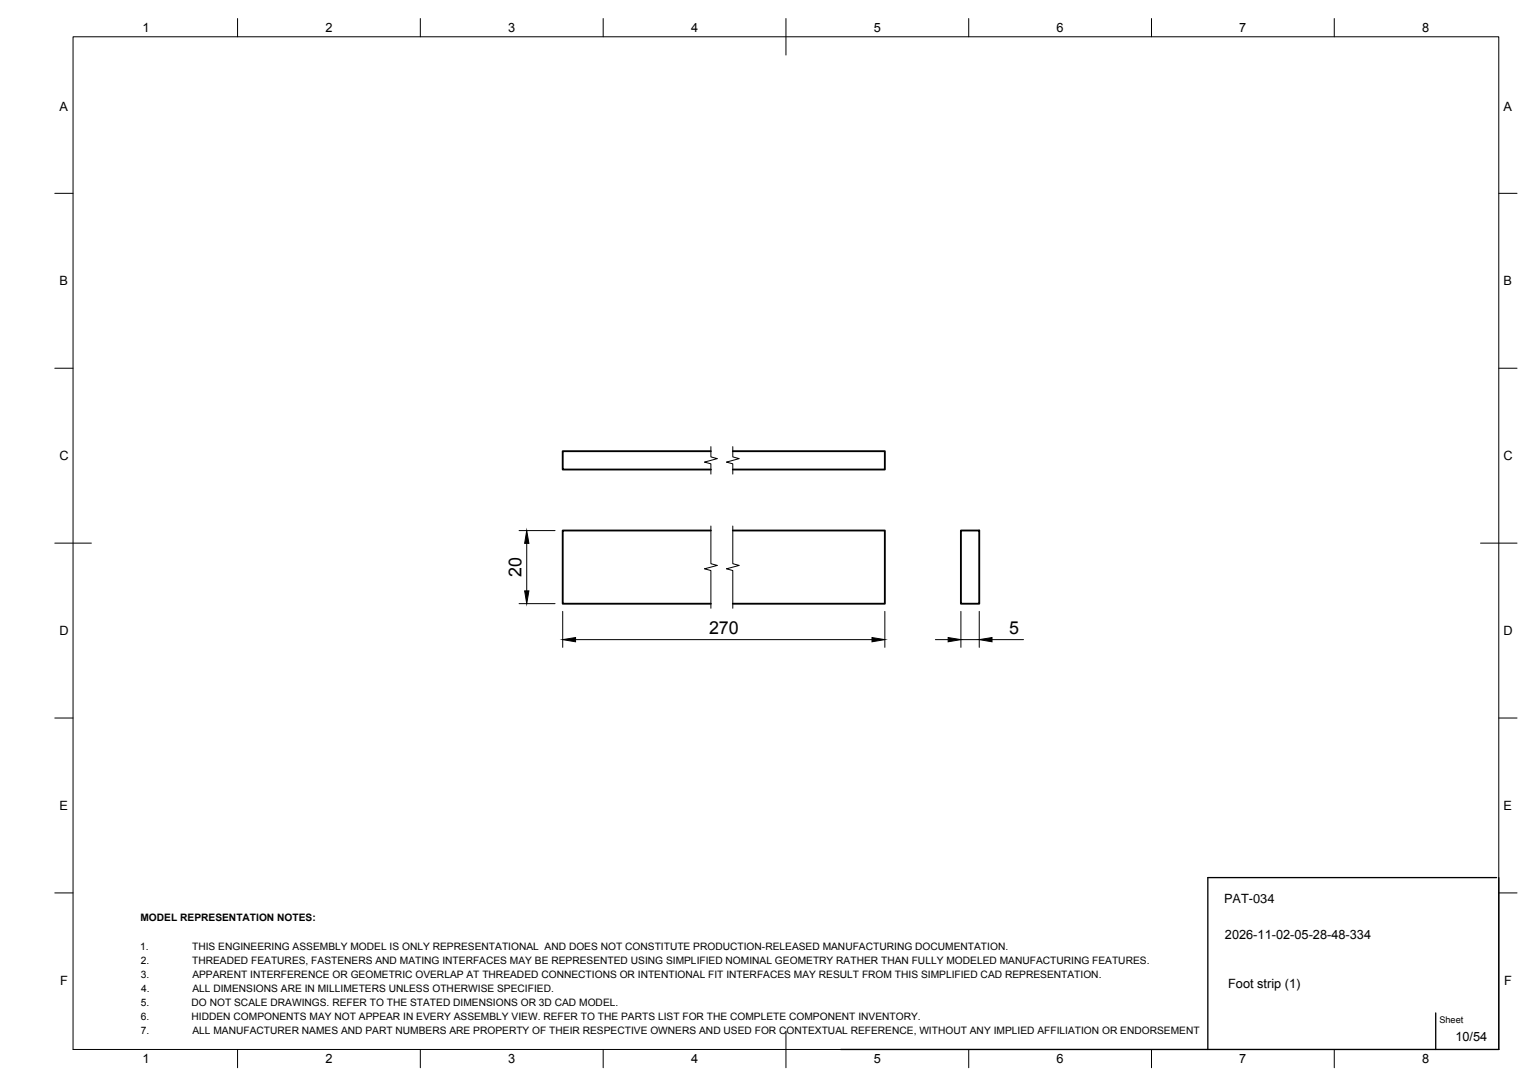
ISO-10303-21;
HEADER;
/* Generated by software containing ST-Developer
 * from STEP Tools, Inc. (www.steptools.com) 
 */

FILE_DESCRIPTION(
/* description */ ('Fatigue rig crank-slider'),
/* implementation_level */ '2;1');

FILE_NAME(
/* name */ 'Foot strip (1).step',
/* time_stamp */ '2026-10-28T03:24:50-07:00',
/* author */ (''),
/* organization */ (''),
/* preprocessor_version */ 'ST-DEVELOPER v20.2',
/* originating_system */ 'Autodesk Translation Framework v15.17.0.0',
/* authorisation */ '');

FILE_SCHEMA (('AUTOMOTIVE_DESIGN { 1 0 10303 214 3 1 1 }'));
ENDSEC;

DATA;
#10=MECHANICAL_DESIGN_GEOMETRIC_PRESENTATION_REPRESENTATION('',(#596),#16911);
#496=SHAPE_REPRESENTATION_RELATIONSHIP('SRR','None',#17135,#546);
#546=ADVANCED_BREP_SHAPE_REPRESENTATION('',(#655),#16864);
#596=STYLED_ITEM('',(#17473),#655);
#655=MANIFOLD_SOLID_BREP('Body1',#8887);
#955=PLANE('',#9719);
#956=PLANE('',#9720);
#957=PLANE('',#9721);
#958=PLANE('',#9722);
#959=PLANE('',#9723);
#960=PLANE('',#9724);
#1327=FACE_OUTER_BOUND('',#1926,.T.);
#1328=FACE_OUTER_BOUND('',#1927,.T.);
#1329=FACE_OUTER_BOUND('',#1928,.T.);
#1330=FACE_OUTER_BOUND('',#1929,.T.);
#1331=FACE_OUTER_BOUND('',#1930,.T.);
#1332=FACE_OUTER_BOUND('',#1931,.T.);
#1926=EDGE_LOOP('',(#6428,#6429,#6430,#6431));
#1927=EDGE_LOOP('',(#6432,#6433,#6434,#6435));
#1928=EDGE_LOOP('',(#6436,#6437,#6438,#6439));
#1929=EDGE_LOOP('',(#6440,#6441,#6442,#6443));
#1930=EDGE_LOOP('',(#6444,#6445,#6446,#6447));
#1931=EDGE_LOOP('',(#6448,#6449,#6450,#6451));
#2572=LINE('',#13843,#3218);
#2573=LINE('',#13845,#3219);
#2574=LINE('',#13847,#3220);
#2575=LINE('',#13848,#3221);
#2576=LINE('',#13851,#3222);
#2577=LINE('',#13853,#3223);
#2578=LINE('',#13854,#3224);
#2579=LINE('',#13857,#3225);
#2580=LINE('',#13859,#3226);
#2581=LINE('',#13860,#3227);
#2582=LINE('',#13862,#3228);
#2583=LINE('',#13863,#3229);
#3218=VECTOR('',#11132,1.);
#3219=VECTOR('',#11133,1.);
#3220=VECTOR('',#11134,1.);
#3221=VECTOR('',#11135,1.);
#3222=VECTOR('',#11138,1.);
#3223=VECTOR('',#11139,1.);
#3224=VECTOR('',#11140,1.);
#3225=VECTOR('',#11143,1.);
#3226=VECTOR('',#11144,1.);
#3227=VECTOR('',#11145,1.);
#3228=VECTOR('',#11148,1.);
#3229=VECTOR('',#11149,1.);
#4296=VERTEX_POINT('',#13841);
#4297=VERTEX_POINT('',#13842);
#4298=VERTEX_POINT('',#13844);
#4299=VERTEX_POINT('',#13846);
#4300=VERTEX_POINT('',#13850);
#4301=VERTEX_POINT('',#13852);
#4302=VERTEX_POINT('',#13856);
#4303=VERTEX_POINT('',#13858);
#5112=EDGE_CURVE('',#4296,#4297,#2572,.T.);
#5113=EDGE_CURVE('',#4297,#4298,#2573,.T.);
#5114=EDGE_CURVE('',#4299,#4298,#2574,.T.);
#5115=EDGE_CURVE('',#4296,#4299,#2575,.T.);
#5116=EDGE_CURVE('',#4300,#4296,#2576,.T.);
#5117=EDGE_CURVE('',#4301,#4299,#2577,.T.);
#5118=EDGE_CURVE('',#4300,#4301,#2578,.T.);
#5119=EDGE_CURVE('',#4302,#4300,#2579,.T.);
#5120=EDGE_CURVE('',#4303,#4301,#2580,.T.);
#5121=EDGE_CURVE('',#4302,#4303,#2581,.T.);
#5122=EDGE_CURVE('',#4297,#4302,#2582,.T.);
#5123=EDGE_CURVE('',#4298,#4303,#2583,.T.);
#6428=ORIENTED_EDGE('',*,*,#5112,.T.);
#6429=ORIENTED_EDGE('',*,*,#5113,.T.);
#6430=ORIENTED_EDGE('',*,*,#5114,.F.);
#6431=ORIENTED_EDGE('',*,*,#5115,.F.);
#6432=ORIENTED_EDGE('',*,*,#5116,.T.);
#6433=ORIENTED_EDGE('',*,*,#5115,.T.);
#6434=ORIENTED_EDGE('',*,*,#5117,.F.);
#6435=ORIENTED_EDGE('',*,*,#5118,.F.);
#6436=ORIENTED_EDGE('',*,*,#5119,.T.);
#6437=ORIENTED_EDGE('',*,*,#5118,.T.);
#6438=ORIENTED_EDGE('',*,*,#5120,.F.);
#6439=ORIENTED_EDGE('',*,*,#5121,.F.);
#6440=ORIENTED_EDGE('',*,*,#5122,.T.);
#6441=ORIENTED_EDGE('',*,*,#5121,.T.);
#6442=ORIENTED_EDGE('',*,*,#5123,.F.);
#6443=ORIENTED_EDGE('',*,*,#5113,.F.);
#6444=ORIENTED_EDGE('',*,*,#5123,.T.);
#6445=ORIENTED_EDGE('',*,*,#5120,.T.);
#6446=ORIENTED_EDGE('',*,*,#5117,.T.);
#6447=ORIENTED_EDGE('',*,*,#5114,.T.);
#6448=ORIENTED_EDGE('',*,*,#5122,.F.);
#6449=ORIENTED_EDGE('',*,*,#5112,.F.);
#6450=ORIENTED_EDGE('',*,*,#5116,.F.);
#6451=ORIENTED_EDGE('',*,*,#5119,.F.);
#8465=ADVANCED_FACE('',(#1327),#955,.T.);
#8466=ADVANCED_FACE('',(#1328),#956,.T.);
#8467=ADVANCED_FACE('',(#1329),#957,.T.);
#8468=ADVANCED_FACE('',(#1330),#958,.T.);
#8469=ADVANCED_FACE('',(#1331),#959,.T.);
#8470=ADVANCED_FACE('',(#1332),#960,.F.);
#8887=CLOSED_SHELL('',(#8465,#8466,#8467,#8468,#8469,#8470));
#9718=AXIS2_PLACEMENT_3D('',#13839,#11128,#11129);
#9719=AXIS2_PLACEMENT_3D('',#13840,#11130,#11131);
#9720=AXIS2_PLACEMENT_3D('',#13849,#11136,#11137);
#9721=AXIS2_PLACEMENT_3D('',#13855,#11141,#11142);
#9722=AXIS2_PLACEMENT_3D('',#13861,#11146,#11147);
#9723=AXIS2_PLACEMENT_3D('',#13864,#11150,#11151);
#9724=AXIS2_PLACEMENT_3D('',#13865,#11152,#11153);
#11128=DIRECTION('axis',(0.,0.,1.));
#11129=DIRECTION('refdir',(1.,0.,0.));
#11130=DIRECTION('center_axis',(0.,1.,0.));
#11131=DIRECTION('ref_axis',(-1.,0.,0.));
#11132=DIRECTION('',(-1.,0.,0.));
#11133=DIRECTION('',(0.,0.,1.));
#11134=DIRECTION('',(-1.,0.,0.));
#11135=DIRECTION('',(0.,0.,1.));
#11136=DIRECTION('center_axis',(1.,0.,0.));
#11137=DIRECTION('ref_axis',(0.,1.,0.));
#11138=DIRECTION('',(0.,1.,0.));
#11139=DIRECTION('',(0.,1.,0.));
#11140=DIRECTION('',(0.,0.,1.));
#11141=DIRECTION('center_axis',(0.,-1.,0.));
#11142=DIRECTION('ref_axis',(1.,0.,0.));
#11143=DIRECTION('',(1.,0.,0.));
#11144=DIRECTION('',(1.,0.,0.));
#11145=DIRECTION('',(0.,0.,1.));
#11146=DIRECTION('center_axis',(-1.,0.,0.));
#11147=DIRECTION('ref_axis',(0.,-1.,0.));
#11148=DIRECTION('',(0.,-1.,0.));
#11149=DIRECTION('',(0.,-1.,0.));
#11150=DIRECTION('center_axis',(0.,0.,1.));
#11151=DIRECTION('ref_axis',(1.,0.,0.));
#11152=DIRECTION('center_axis',(0.,0.,1.));
#11153=DIRECTION('ref_axis',(1.,0.,0.));
#13839=CARTESIAN_POINT('',(0.,0.,0.));
#13840=CARTESIAN_POINT('Origin',(24.,9.,-0.5));
#13841=CARTESIAN_POINT('',(24.,9.,-0.5));
#13842=CARTESIAN_POINT('',(22.,9.,-0.5));
#13843=CARTESIAN_POINT('',(24.,9.,-0.5));
#13844=CARTESIAN_POINT('',(22.,9.,0.));
#13845=CARTESIAN_POINT('',(22.,9.,-0.5));
#13846=CARTESIAN_POINT('',(24.,9.,0.));
#13847=CARTESIAN_POINT('',(24.,9.,0.));
#13848=CARTESIAN_POINT('',(24.,9.,-0.5));
#13849=CARTESIAN_POINT('Origin',(24.,-18.,-0.5));
#13850=CARTESIAN_POINT('',(24.,-18.,-0.5));
#13851=CARTESIAN_POINT('',(24.,-18.,-0.5));
#13852=CARTESIAN_POINT('',(24.,-18.,0.));
#13853=CARTESIAN_POINT('',(24.,-18.,0.));
#13854=CARTESIAN_POINT('',(24.,-18.,-0.5));
#13855=CARTESIAN_POINT('Origin',(22.,-18.,-0.5));
#13856=CARTESIAN_POINT('',(22.,-18.,-0.5));
#13857=CARTESIAN_POINT('',(22.,-18.,-0.5));
#13858=CARTESIAN_POINT('',(22.,-18.,0.));
#13859=CARTESIAN_POINT('',(22.,-18.,0.));
#13860=CARTESIAN_POINT('',(22.,-18.,-0.5));
#13861=CARTESIAN_POINT('Origin',(22.,9.,-0.5));
#13862=CARTESIAN_POINT('',(22.,9.,-0.5));
#13863=CARTESIAN_POINT('',(22.,9.,0.));
#13864=CARTESIAN_POINT('Origin',(23.,-4.5,0.));
#13865=CARTESIAN_POINT('Origin',(23.,-4.5,-0.5));
#16805=UNCERTAINTY_MEASURE_WITH_UNIT(LENGTH_MEASURE(0.001),#16912,
'DISTANCE_ACCURACY_VALUE',
'Maximum model space distance between geometric entities at asserted c
onnectivities');
#16852=UNCERTAINTY_MEASURE_WITH_UNIT(LENGTH_MEASURE(0.001),#16912,
'DISTANCE_ACCURACY_VALUE',
'Maximum model space distance between geometric entities at asserted c
onnectivities');
#16864=(
GEOMETRIC_REPRESENTATION_CONTEXT(3)
GLOBAL_UNCERTAINTY_ASSIGNED_CONTEXT((#16805))
GLOBAL_UNIT_ASSIGNED_CONTEXT((#16912,#16914,#16915))
REPRESENTATION_CONTEXT('','3D')
);
#16911=(
GEOMETRIC_REPRESENTATION_CONTEXT(3)
GLOBAL_UNCERTAINTY_ASSIGNED_CONTEXT((#16852))
GLOBAL_UNIT_ASSIGNED_CONTEXT((#16912,#16914,#16915))
REPRESENTATION_CONTEXT('','3D')
);
#16912=(
LENGTH_UNIT()
NAMED_UNIT(*)
SI_UNIT(.CENTI.,.METRE.)
);
#16914=(
NAMED_UNIT(*)
PLANE_ANGLE_UNIT()
SI_UNIT($,.RADIAN.)
);
#16915=(
NAMED_UNIT(*)
SI_UNIT($,.STERADIAN.)
SOLID_ANGLE_UNIT()
);
#16927=SHAPE_DEFINITION_REPRESENTATION(#16985,#17135);
#16985=PRODUCT_DEFINITION_SHAPE('',$,#17194);
#17135=SHAPE_REPRESENTATION('',(#9718),#16864);
#17182=PRODUCT_DEFINITION_CONTEXT('part definition',#17358,'design');
#17194=PRODUCT_DEFINITION('Foot strip (1)','Foot strip (1)',#17252,#17182);
#17252=PRODUCT_DEFINITION_FORMATION('',$,#17371);
#17358=APPLICATION_CONTEXT(
'Core Data for Automotive Mechanical Design Process');
#17359=PRODUCT_CONTEXT('part definition',#17358,'mechanical');
#17371=PRODUCT('Foot strip (1)','Foot strip (1)','Foot strip (1)',(#17359));
#17467=COLOUR_RGB('Light Blue',0.38,0.62,0.78);
#17468=FILL_AREA_STYLE_COLOUR('',#17467);
#17469=FILL_AREA_STYLE('',(#17468));
#17470=SURFACE_STYLE_FILL_AREA(#17469);
#17471=SURFACE_SIDE_STYLE('',(#17470));
#17472=SURFACE_STYLE_USAGE(.BOTH.,#17471);
#17473=PRESENTATION_STYLE_ASSIGNMENT((#17472));
ENDSEC;
END-ISO-10303-21;
